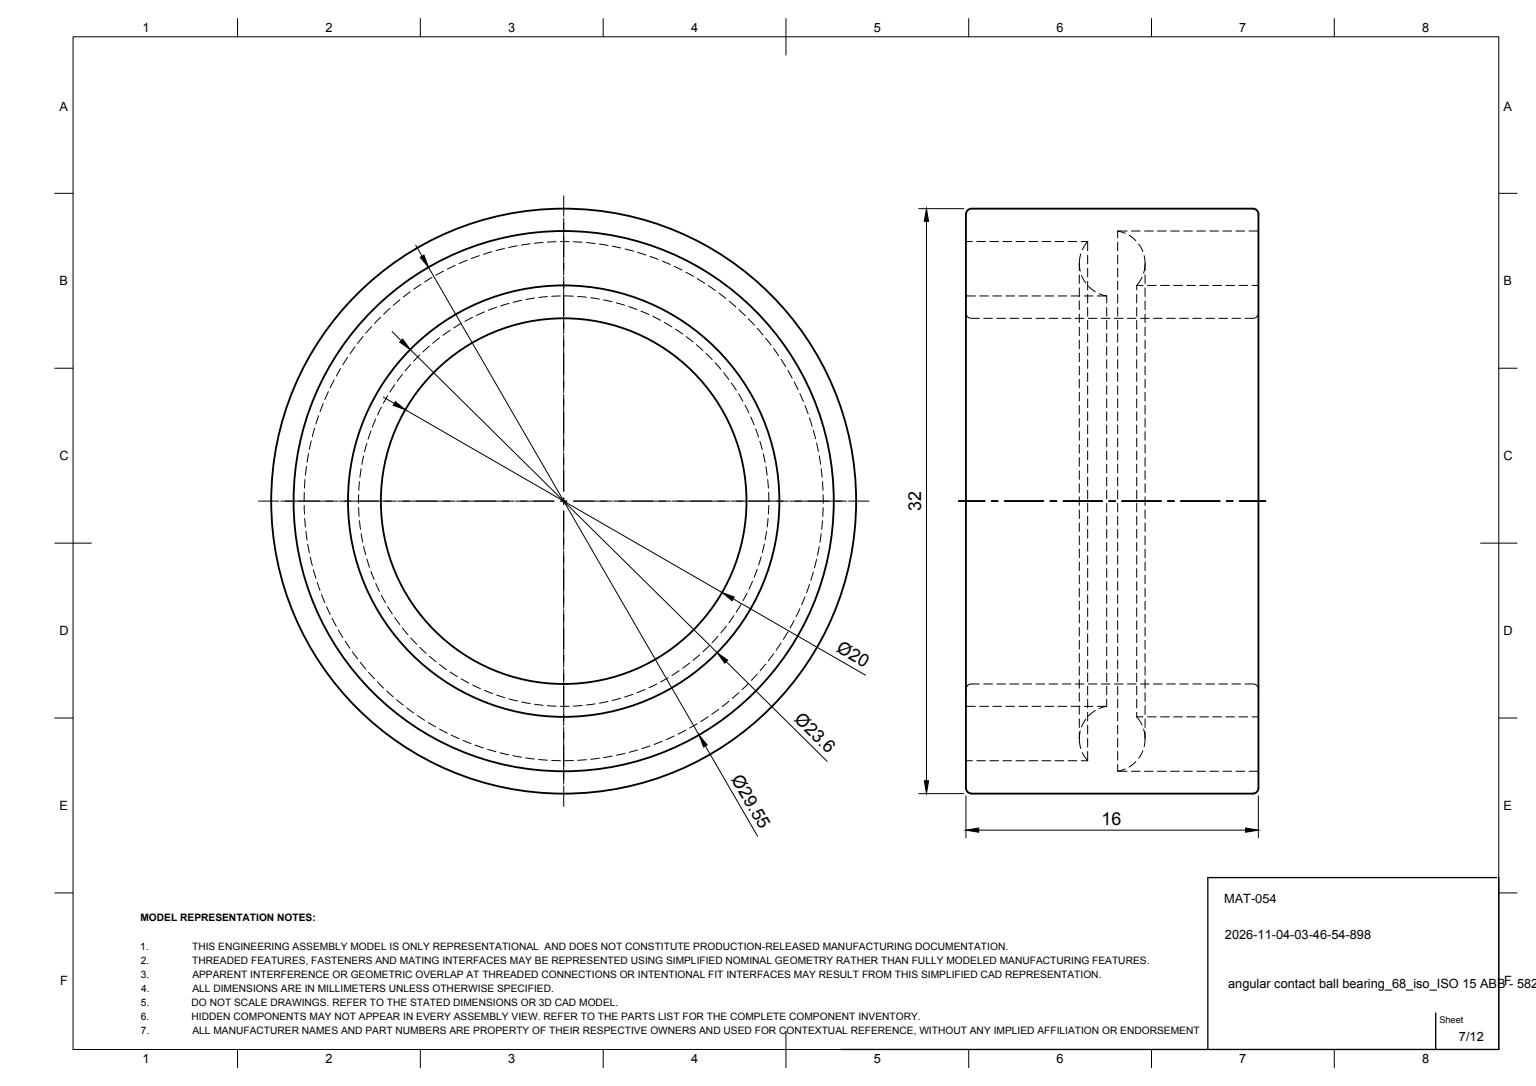
ISO-10303-21;
HEADER;
FILE_DESCRIPTION (('STEP AP214'),
    '1' );
FILE_NAME ('angular contact ball bearing_68_iso_ISO 15 ABB - 5820 - Full,SI,NC,Full_68.step',
    '2026-10-21T17:50:41',
    ( '' ),
    ( '' ),
    'SwSTEP 2.0',
    'SolidWorks 2026',
    '' );
FILE_SCHEMA (( 'AUTOMOTIVE_DESIGN' ));
ENDSEC;

DATA;
#7=EDGE_CURVE ( 'NONE', #6804, #14714, #31558, .T. ) ;
#8=ADVANCED_FACE ( 'NONE', ( #33361 ), #14697, .F. ) ;
#38=PLANE ( 'NONE',  #8347 ) ;
#124=LINE ( 'NONE', #5791, #25297 ) ;
#171=EDGE_CURVE ( 'NONE', #17976, #25124, #32703, .T. ) ;
#186=CARTESIAN_POINT ( 'NONE',  ( 8.000000000000000000, 0.000000000000000000, -14.19999999999999929 ) ) ;
#233=PRODUCT_DEFINITION_FORMATION_WITH_SPECIFIED_SOURCE ( 'ANY', '', #8627, .NOT_KNOWN. ) ;
#246=CARTESIAN_POINT ( 'NONE',  ( 8.000000000000000000, 0.000000000000000000, -15.69999999999999929 ) ) ;
#264=DIRECTION ( 'NONE',  ( 1.000000000000000000, 0.000000000000000000, 0.000000000000000000 ) ) ;
#277=EDGE_CURVE ( 'NONE', #32572, #17435, #29890, .T. ) ;
#329=PRODUCT_DEFINITION ( 'UNKNOWN', '', #233, #29569 ) ;
#379=ORIENTED_EDGE ( 'NONE', *, *, #10888, .T. ) ;
#466=CARTESIAN_POINT ( 'NONE',  ( -0.2989565185775304723, 0.000000000000000000, 0.000000000000000000 ) ) ;
#469=VERTEX_POINT ( 'NONE', #17506 ) ;
#486=AXIS2_PLACEMENT_3D ( 'NONE', #4593, #26151, #10139 ) ;
#668=DIRECTION ( 'NONE',  ( 0.000000000000000000, 0.000000000000000000, -1.000000000000000000 ) ) ;
#744=DIRECTION ( 'NONE',  ( 1.000000000000000000, 0.000000000000000000, 0.000000000000000000 ) ) ;
#769=VERTEX_POINT ( 'NONE', #186 ) ;
#855=EDGE_CURVE ( 'NONE', #32236, #2476, #6011, .T. ) ;
#998=FACE_OUTER_BOUND ( 'NONE', #9441, .T. ) ;
#1009=CARTESIAN_POINT ( 'NONE',  ( -8.000000000000000000, 0.000000000000000000, -15.69999999999999929 ) ) ;
#1061=ORIENTED_EDGE ( 'NONE', *, *, #9092, .F. ) ;
#1105=CARTESIAN_POINT ( 'NONE',  ( -8.000000000000000000, 0.000000000000000000, 0.000000000000000000 ) ) ;
#1140=FACE_OUTER_BOUND ( 'NONE', #5912, .T. ) ;
#1220=CARTESIAN_POINT ( 'NONE',  ( 0.2989565185775198697, 0.000000000000000000, 11.22499999999999787 ) ) ;
#1314=DIRECTION ( 'NONE',  ( 1.000000000000000000, 0.000000000000000000, 0.000000000000000000 ) ) ;
#1338=AXIS2_PLACEMENT_3D ( 'NONE', #14468, #8753, #12149 ) ;
#1470=ORIENTED_EDGE ( 'NONE', *, *, #32484, .T. ) ;
#1474=ORIENTED_EDGE ( 'NONE', *, *, #5517, .F. ) ;
#1512=ORIENTED_EDGE ( 'NONE', *, *, #16791, .T. ) ;
#1621=CIRCLE ( 'NONE', #19248, 16.00000000000000000 ) ;
#1632=EDGE_LOOP ( 'NONE', ( #11200, #2339 ) ) ;
#1652=LINE ( 'NONE', #10193, #28394 ) ;
#1666=CARTESIAN_POINT ( 'NONE',  ( 8.000000000000000000, 0.000000000000000000, 0.000000000000000000 ) ) ;
#1759=DIRECTION ( 'NONE',  ( 0.000000000000000000, 0.000000000000000000, -1.000000000000000000 ) ) ;
#1870=VERTEX_POINT ( 'NONE', #7097 ) ;
#1930=FACE_OUTER_BOUND ( 'NONE', #28195, .T. ) ;
#1931=CARTESIAN_POINT ( 'NONE',  ( -20.63749999999999929, 0.000000000000000000, 0.000000000000000000 ) ) ;
#1947=EDGE_CURVE ( 'NONE', #32236, #1870, #22836, .T. ) ;
#1949=ADVANCED_FACE ( 'NONE', ( #3780 ), #17900, .T. ) ;
#1989=DIRECTION ( 'NONE',  ( 0.000000000000000000, 1.000000000000000000, -1.224646799147353207E-16 ) ) ;
#2151=CYLINDRICAL_SURFACE ( 'NONE', #19584, 16.00000000000000000 ) ;
#2172=ORIENTED_EDGE ( 'NONE', *, *, #16791, .F. ) ;
#2200=DIRECTION ( 'NONE',  ( 0.000000000000000000, 0.000000000000000000, 1.000000000000000000 ) ) ;
#2203=ORIENTED_EDGE ( 'NONE', *, *, #4582, .F. ) ;
#2226=DIRECTION ( 'NONE',  ( 0.000000000000000000, -1.000000000000000000, 0.000000000000000000 ) ) ;
#2240=AXIS2_PLACEMENT_3D ( 'NONE', #7866, #23538, #34222 ) ;
#2314=CYLINDRICAL_SURFACE ( 'NONE', #26398, 11.22499999999999787 ) ;
#2339=ORIENTED_EDGE ( 'NONE', *, *, #22792, .T. ) ;
#2356=DIRECTION ( 'NONE',  ( 0.000000000000000000, 0.000000000000000000, -1.000000000000000000 ) ) ;
#2388=CARTESIAN_POINT ( 'NONE',  ( 8.000000000000000000, 0.000000000000000000, 0.000000000000000000 ) ) ;
#2463=CARTESIAN_POINT ( 'NONE',  ( 7.700000000000000178, 0.000000000000000000, 0.000000000000000000 ) ) ;
#2476=VERTEX_POINT ( 'NONE', #4551 ) ;
#2563=FACE_OUTER_BOUND ( 'NONE', #29011, .T. ) ;
#2569=FACE_OUTER_BOUND ( 'NONE', #17868, .T. ) ;
#2634=AXIS2_PLACEMENT_3D ( 'NONE', #24105, #26962, #27301 ) ;
#2700=CARTESIAN_POINT ( 'NONE',  ( 8.000000000000000000, 0.000000000000000000, 0.000000000000000000 ) ) ;
#2704=DIRECTION ( 'NONE',  ( 0.000000000000000000, 0.000000000000000000, 1.000000000000000000 ) ) ;
#2713=CARTESIAN_POINT ( 'NONE',  ( -1.341640786499875171, 0.000000000000000000, 0.000000000000000000 ) ) ;
#2745=CYLINDRICAL_SURFACE ( 'NONE', #15332, 16.00000000000000000 ) ;
#2757=EDGE_CURVE ( 'NONE', #30850, #6804, #4173, .T. ) ;
#2803=DIRECTION ( 'NONE',  ( 0.000000000000000000, 1.000000000000000000, -1.224646799147353207E-16 ) ) ;
#2837=CARTESIAN_POINT ( 'NONE',  ( 1.341640786499872284, 0.000000000000000000, 0.000000000000000000 ) ) ;
#2846=DIRECTION ( 'NONE',  ( 1.000000000000000000, 0.000000000000000000, 0.000000000000000000 ) ) ;
#2912=CARTESIAN_POINT ( 'NONE',  ( 7.699999999999998401, 0.000000000000000000, 0.000000000000000000 ) ) ;
#2946=DIRECTION ( 'NONE',  ( 1.000000000000000000, 0.000000000000000000, 0.000000000000000000 ) ) ;
#3184=CARTESIAN_POINT ( 'NONE',  ( -7.700000000000000178, 0.000000000000000000, -16.00000000000000000 ) ) ;
#3194=CARTESIAN_POINT ( 'NONE',  ( 7.699999999999998401, 1.959434878635765131E-15, 16.00000000000000000 ) ) ;
#3197=DIRECTION ( 'NONE',  ( 0.000000000000000000, -1.224646799147353454E-16, 1.000000000000000000 ) ) ;
#3275=ORIENTED_EDGE ( 'NONE', *, *, #1947, .F. ) ;
#3330=DIRECTION ( 'NONE',  ( 1.000000000000000000, 0.000000000000000000, 0.000000000000000000 ) ) ;
#3367=DIRECTION ( 'NONE',  ( 0.000000000000000000, 1.224646799147346305E-16, 1.000000000000000000 ) ) ;
#3373=CIRCLE ( 'NONE', #11906, 15.69999999999999929 ) ;
#3511=PLANE ( 'NONE',  #20460 ) ;
#3593=EDGE_CURVE ( 'NONE', #13790, #9326, #20313, .T. ) ;
#3597=TOROIDAL_SURFACE ( 'NONE', #22389, 10.30000000000000071, 0.3000000000000025424 ) ;
#3622=CARTESIAN_POINT ( 'NONE',  ( 7.700000000000001954, 1.243016501134563095E-15, 9.999999999999994671 ) ) ;
#3674=CARTESIAN_POINT ( 'NONE',  ( 8.000000000000000000, 0.000000000000000000, 0.000000000000000000 ) ) ;
#3756=ORIENTED_EDGE ( 'NONE', *, *, #29048, .T. ) ;
#3780=FACE_OUTER_BOUND ( 'NONE', #21252, .T. ) ;
#3795=TOROIDAL_SURFACE ( 'NONE', #27678, 15.69999999999999929, 0.3000000000000007661 ) ;
#3891=TOROIDAL_SURFACE ( 'NONE', #34624, 13.00000000000000000, 1.799999999999999822 ) ;
#3911=TOROIDAL_SURFACE ( 'NONE', #29521, 10.30000000000000071, 0.3000000000000025424 ) ;
#3937=DIRECTION ( 'NONE',  ( 0.000000000000000000, 0.000000000000000000, -1.000000000000000000 ) ) ;
#3990=CIRCLE ( 'NONE', #21637, 1.799999999999999600 ) ;
#4004=FACE_OUTER_BOUND ( 'NONE', #29965, .T. ) ;
#4173=LINE ( 'NONE', #15062, #12299 ) ;
#4194=ORIENTED_EDGE ( 'NONE', *, *, #13037, .T. ) ;
#4241=ADVANCED_FACE ( 'NONE', ( #2563, #31592 ), #7197, .T. ) ;
#4258=TOROIDAL_SURFACE ( 'NONE', #29276, 10.30000000000000071, 0.3000000000000025424 ) ;
#4300=EDGE_LOOP ( 'NONE', ( #16936, #7458, #13111, #5106 ) ) ;
#4312=FACE_OUTER_BOUND ( 'NONE', #33109, .T. ) ;
#4387=CARTESIAN_POINT ( 'NONE',  ( 0.000000000000000000, 0.000000000000000000, 13.00000000000000000 ) ) ;
#4441=CARTESIAN_POINT ( 'NONE',  ( 0.000000000000000000, 1.592040838891559095E-15, -13.00000000000000000 ) ) ;
#4481=ORIENTED_EDGE ( 'NONE', *, *, #29502, .F. ) ;
#4551=CARTESIAN_POINT ( 'NONE',  ( 1.341640786499872284, 1.738998454789241944E-15, -14.20000000000000107 ) ) ;
#4582=EDGE_CURVE ( 'NONE', #22453, #23243, #1652, .T. ) ;
#4593=CARTESIAN_POINT ( 'NONE',  ( 8.000000000000000000, 0.000000000000000000, 0.000000000000000000 ) ) ;
#4623=EDGE_CURVE ( 'NONE', #23243, #30812, #17619, .T. ) ;
#4650=EDGE_LOOP ( 'NONE', ( #32477, #31030, #19102, #11073 ) ) ;
#4704=DIRECTION ( 'NONE',  ( 0.000000000000000000, 0.000000000000000000, -1.000000000000000000 ) ) ;
#4727=DIRECTION ( 'NONE',  ( 1.000000000000000000, 0.000000000000000000, 0.000000000000000000 ) ) ;
#4773=VECTOR ( 'NONE', #4727, 1000.000000000000000 ) ;
#4787=ORIENTED_EDGE ( 'NONE', *, *, #277, .T. ) ;
#4819=ORIENTED_EDGE ( 'NONE', *, *, #29048, .F. ) ;
#4833=DIRECTION ( 'NONE',  ( 1.000000000000000000, 0.000000000000000000, 0.000000000000000000 ) ) ;
#4852=DIRECTION ( 'NONE',  ( 0.000000000000000000, 0.000000000000000000, -1.000000000000000000 ) ) ;
#4894=( NAMED_UNIT ( * ) SI_UNIT ( $, .STERADIAN. ) SOLID_ANGLE_UNIT ( ) );
#4946=CYLINDRICAL_SURFACE ( 'NONE', #12641, 11.80000000000000071 ) ;
#4981=VECTOR ( 'NONE', #744, 1000.000000000000000 ) ;
#5004=CIRCLE ( 'NONE', #24905, 10.30000000000000071 ) ;
#5033=DIRECTION ( 'NONE',  ( 1.000000000000000000, 0.000000000000000000, 0.000000000000000000 ) ) ;
#5086=CARTESIAN_POINT ( 'NONE',  ( -20.63749999999999929, 1.445083222993876839E-15, 11.80000000000000071 ) ) ;
#5106=ORIENTED_EDGE ( 'NONE', *, *, #13037, .F. ) ;
#5174=ORIENTED_EDGE ( 'NONE', *, *, #33517, .F. ) ;
#5178=DIRECTION ( 'NONE',  ( 0.000000000000000000, 0.000000000000000000, -1.000000000000000000 ) ) ;
#5226=DIRECTION ( 'NONE',  ( 1.000000000000000000, 0.000000000000000000, 0.000000000000000000 ) ) ;
#5295=ORIENTED_EDGE ( 'NONE', *, *, #1947, .T. ) ;
#5306=ORIENTED_EDGE ( 'NONE', *, *, #14522, .F. ) ;
#5332=CARTESIAN_POINT ( 'NONE',  ( -8.000000000000000000, 0.000000000000000000, 0.000000000000000000 ) ) ;
#5350=AXIS2_PLACEMENT_3D ( 'NONE', #23000, #33497, #25484 ) ;
#5395=ORIENTED_EDGE ( 'NONE', *, *, #17447, .F. ) ;
#5517=EDGE_CURVE ( 'NONE', #14714, #6804, #6686, .T. ) ;
#5585=DIRECTION ( 'NONE',  ( 0.000000000000000000, 0.000000000000000000, -1.000000000000000000 ) ) ;
#5589=DIRECTION ( 'NONE',  ( 1.000000000000000000, 0.000000000000000000, 0.000000000000000000 ) ) ;
#5616=DIRECTION ( 'NONE',  ( 1.000000000000000000, 0.000000000000000000, 0.000000000000000000 ) ) ;
#5668=ORIENTED_EDGE ( 'NONE', *, *, #22792, .F. ) ;
#5727=STYLED_ITEM('',(#35275),#33706);
#5729=ORIENTED_EDGE ( 'NONE', *, *, #20886, .T. ) ;
#5752=AXIS2_PLACEMENT_3D ( 'NONE', #5332, #16223, #27229 ) ;
#5761=VERTEX_POINT ( 'NONE', #15409 ) ;
#5791=CARTESIAN_POINT ( 'NONE',  ( -20.63749999999999929, 1.374666032042903655E-15, 11.22499999999999787 ) ) ;
#5813=EDGE_CURVE ( 'NONE', #15484, #32236, #12770, .T. ) ;
#5828=CIRCLE ( 'NONE', #18942, 0.3000000000000016542 ) ;
#5912=EDGE_LOOP ( 'NONE', ( #4819, #28442, #12506, #24370 ) ) ;
#6011=CIRCLE ( 'NONE', #35032, 1.799999999999999600 ) ;
#6047=SHAPE_DEFINITION_REPRESENTATION ( #6066, #19821 ) ;
#6052=CARTESIAN_POINT ( 'NONE',  ( 0.2989565185775198697, 0.000000000000000000, 0.000000000000000000 ) ) ;
#6063=LINE ( 'NONE', #13924, #4981 ) ;
#6066=PRODUCT_DEFINITION_SHAPE ( 'NONE', 'NONE',  #329 ) ;
#6110=DIRECTION ( 'NONE',  ( 1.000000000000000000, 0.000000000000000000, 0.000000000000000000 ) ) ;
#6201=DIRECTION ( 'NONE',  ( 0.000000000000000000, 1.000000000000000000, -1.224646799147353207E-16 ) ) ;
#6256=( NAMED_UNIT ( * ) PLANE_ANGLE_UNIT ( ) SI_UNIT ( $, .RADIAN. ) );
#6272=AXIS2_PLACEMENT_3D ( 'NONE', #2388, #13971, #32981 ) ;
#6314=AXIS2_PLACEMENT_3D ( 'NONE', #14281, #24931, #11421 ) ;
#6323=DIRECTION ( 'NONE',  ( 1.000000000000000000, 0.000000000000000000, 0.000000000000000000 ) ) ;
#6375=DIRECTION ( 'NONE',  ( 0.000000000000000000, 0.000000000000000000, -1.000000000000000000 ) ) ;
#6392=ORIENTED_EDGE ( 'NONE', *, *, #9137, .F. ) ;
#6393=CIRCLE ( 'NONE', #21163, 11.79999999999999893 ) ;
#6423=DIRECTION ( 'NONE',  ( 1.000000000000000000, 0.000000000000000000, 0.000000000000000000 ) ) ;
#6595=DIRECTION ( 'NONE',  ( 1.000000000000000000, 0.000000000000000000, 0.000000000000000000 ) ) ;
#6686=CIRCLE ( 'NONE', #17519, 14.77500000000000036 ) ;
#6700=ORIENTED_EDGE ( 'NONE', *, *, #21011, .F. ) ;
#6778=EDGE_CURVE ( 'NONE', #15484, #28564, #124, .T. ) ;
#6804=VERTEX_POINT ( 'NONE', #24847 ) ;
#6851=DIRECTION ( 'NONE',  ( 0.000000000000000000, 0.000000000000000000, 1.000000000000000000 ) ) ;
#6867=ADVANCED_FACE ( 'NONE', ( #4004 ), #32690, .T. ) ;
#6922=DIRECTION ( 'NONE',  ( 1.000000000000000000, 0.000000000000000000, 0.000000000000000000 ) ) ;
#6953=AXIS2_PLACEMENT_3D ( 'NONE', #28762, #23774, #4704 ) ;
#7044=CYLINDRICAL_SURFACE ( 'NONE', #9762, 9.999999999999996447 ) ;
#7063=ORIENTED_EDGE ( 'NONE', *, *, #9331, .F. ) ;
#7086=DIRECTION ( 'NONE',  ( 1.000000000000000000, 0.000000000000000000, 0.000000000000000000 ) ) ;
#7097=CARTESIAN_POINT ( 'NONE',  ( 8.000000000000000000, 0.000000000000000000, -11.22499999999999787 ) ) ;
#7155=CARTESIAN_POINT ( 'NONE',  ( -20.63749999999999574, 0.000000000000000000, 0.000000000000000000 ) ) ;
#7197=PLANE ( 'NONE',  #30658 ) ;
#7243=DIRECTION ( 'NONE',  ( 1.000000000000000000, 0.000000000000000000, 0.000000000000000000 ) ) ;
#7281=EDGE_CURVE ( 'NONE', #23878, #9326, #23633, .T. ) ;
#7393=DIRECTION ( 'NONE',  ( 0.000000000000000000, 0.000000000000000000, -1.000000000000000000 ) ) ;
#7458=ORIENTED_EDGE ( 'NONE', *, *, #33947, .T. ) ;
#7508=CARTESIAN_POINT ( 'NONE',  ( 1.341640786499872284, 0.000000000000000000, 0.000000000000000000 ) ) ;
#7534=DIRECTION ( 'NONE',  ( 1.000000000000000000, 0.000000000000000000, 0.000000000000000000 ) ) ;
#7578=DIRECTION ( 'NONE',  ( 0.000000000000000000, 0.000000000000000000, 1.000000000000000000 ) ) ;
#7612=ORIENTED_EDGE ( 'NONE', *, *, #7281, .F. ) ;
#7665=AXIS2_PLACEMENT_3D ( 'NONE', #17019, #17548, #14516 ) ;
#7702=CARTESIAN_POINT ( 'NONE',  ( 0.2989565185775198697, 1.556832243416072701E-15, -11.22499999999999787 ) ) ;
#7731=DIRECTION ( 'NONE',  ( 0.000000000000000000, 0.000000000000000000, -1.000000000000000000 ) ) ;
#7809=APPLICATION_CONTEXT ( 'automotive_design' ) ;
#7813=AXIS2_PLACEMENT_3D ( 'NONE', #11340, #6323, #8651 ) ;
#7866=CARTESIAN_POINT ( 'NONE',  ( 7.700000000000001954, 0.000000000000000000, 0.000000000000000000 ) ) ;
#7867=DIRECTION ( 'NONE',  ( 0.000000000000000000, 0.000000000000000000, -1.000000000000000000 ) ) ;
#7929=ORIENTED_EDGE ( 'NONE', *, *, #33766, .F. ) ;
#7940=DIRECTION ( 'NONE',  ( -1.000000000000000000, -0.000000000000000000, -0.000000000000000000 ) ) ;
#7994=ORIENTED_EDGE ( 'NONE', *, *, #25214, .T. ) ;
#8003=AXIS2_PLACEMENT_3D ( 'NONE', #10952, #5589, #29819 ) ;
#8066=CIRCLE ( 'NONE', #12634, 9.999999999999998224 ) ;
#8114=LINE ( 'NONE', #5086, #4773 ) ;
#8159=ORIENTED_EDGE ( 'NONE', *, *, #12607, .T. ) ;
#8186=CARTESIAN_POINT ( 'NONE',  ( -20.63749999999999929, 0.000000000000000000, 0.000000000000000000 ) ) ;
#8219=CARTESIAN_POINT ( 'NONE',  ( -8.000000000000000000, 11.79999999999999893, 0.000000000000000000 ) ) ;
#8232=CARTESIAN_POINT ( 'NONE',  ( -20.63749999999999929, 0.000000000000000000, 0.000000000000000000 ) ) ;
#8306=CARTESIAN_POINT ( 'NONE',  ( -7.700000000000000178, 0.000000000000000000, 0.000000000000000000 ) ) ;
#8309=DIRECTION ( 'NONE',  ( 1.000000000000000000, 0.000000000000000000, 0.000000000000000000 ) ) ;
#8347=AXIS2_PLACEMENT_3D ( 'NONE', #8219, #19279, #30114 ) ;
#8352=EDGE_CURVE ( 'NONE', #22453, #21269, #15747, .T. ) ;
#8443=ADVANCED_FACE ( 'NONE', ( #34806 ), #32121, .F. ) ;
#8472=CARTESIAN_POINT ( 'NONE',  ( -7.700000000000000178, 0.000000000000000000, 0.000000000000000000 ) ) ;
#8627=PRODUCT ( 'angular contact ball bearing_68_iso_ISO 15 ABB - 5820 - Full,SI,NC,Full_68', 'angular contact ball bearing_68_iso_ISO 15 ABB - 5820 - Full,SI,NC,Full_68', '', ( #25094 ) ) ;
#8651=DIRECTION ( 'NONE',  ( 0.000000000000000000, 0.000000000000000000, -1.000000000000000000 ) ) ;
#8724=ORIENTED_EDGE ( 'NONE', *, *, #34882, .T. ) ;
#8737=EDGE_LOOP ( 'NONE', ( #34351, #34926 ) ) ;
#8742=DIRECTION ( 'NONE',  ( 0.000000000000000000, 0.000000000000000000, -1.000000000000000000 ) ) ;
#8753=DIRECTION ( 'NONE',  ( 0.000000000000000000, -1.000000000000000000, 0.000000000000000000 ) ) ;
#8771=ORIENTED_EDGE ( 'NONE', *, *, #6778, .F. ) ;
#8856=CARTESIAN_POINT ( 'NONE',  ( 7.700000000000000178, 1.261386203121773722E-15, 10.30000000000000071 ) ) ;
#8889=CARTESIAN_POINT ( 'NONE',  ( 7.700000000000000178, 1.922695474661344271E-15, 15.69999999999999929 ) ) ;
#8915=DIRECTION ( 'NONE',  ( -1.000000000000000000, -0.000000000000000000, -0.000000000000000000 ) ) ;
#8939=AXIS2_PLACEMENT_3D ( 'NONE', #30824, #6423, #17321 ) ;
#8972=CARTESIAN_POINT ( 'NONE',  ( -20.63749999999999574, 0.000000000000000000, 0.000000000000000000 ) ) ;
#9007=DIRECTION ( 'NONE',  ( 0.000000000000000000, 0.000000000000000000, -1.000000000000000000 ) ) ;
#9059=CARTESIAN_POINT ( 'NONE',  ( -7.700000000000000178, 0.000000000000000000, 0.000000000000000000 ) ) ;
#9092=EDGE_CURVE ( 'NONE', #5761, #30633, #17839, .T. ) ;
#9137=EDGE_CURVE ( 'NONE', #5761, #469, #16938, .T. ) ;
#9319=DIRECTION ( 'NONE',  ( 1.000000000000000000, 0.000000000000000000, 0.000000000000000000 ) ) ;
#9326=VERTEX_POINT ( 'NONE', #3194 ) ;
#9331=EDGE_CURVE ( 'NONE', #469, #5761, #6393, .T. ) ;
#9441=EDGE_LOOP ( 'NONE', ( #11859, #34213, #13046, #18356 ) ) ;
#9495=ORIENTED_EDGE ( 'NONE', *, *, #17447, .T. ) ;
#9525=EDGE_LOOP ( 'NONE', ( #4787, #8724, #10418, #34158 ) ) ;
#9653=ORIENTED_EDGE ( 'NONE', *, *, #18373, .F. ) ;
#9667=DIRECTION ( 'NONE',  ( 0.000000000000000000, 0.000000000000000000, -1.000000000000000000 ) ) ;
#9728=ADVANCED_FACE ( 'NONE', ( #14262 ), #25090, .T. ) ;
#9762=AXIS2_PLACEMENT_3D ( 'NONE', #28429, #28774, #7393 ) ;
#9811=CIRCLE ( 'NONE', #6953, 0.3000000000000016542 ) ;
#9838=LINE ( 'NONE', #33697, #11415 ) ;
#9871=EDGE_CURVE ( 'NONE', #12372, #21269, #5004, .T. ) ;
#9894=ORIENTED_EDGE ( 'NONE', *, *, #171, .F. ) ;
#9902=ORIENTED_EDGE ( 'NONE', *, *, #7, .F. ) ;
#9903=FACE_OUTER_BOUND ( 'NONE', #34611, .T. ) ;
#9958=CARTESIAN_POINT ( 'NONE',  ( -8.000000000000000000, 0.000000000000000000, 0.000000000000000000 ) ) ;
#10045=VERTEX_POINT ( 'NONE', #18861 ) ;
#10070=ORIENTED_EDGE ( 'NONE', *, *, #17795, .T. ) ;
#10139=DIRECTION ( 'NONE',  ( 0.000000000000000000, 0.000000000000000000, -1.000000000000000000 ) ) ;
#10150=ORIENTED_EDGE ( 'NONE', *, *, #21782, .T. ) ;
#10158=DIRECTION ( 'NONE',  ( 0.000000000000000000, 0.000000000000000000, -1.000000000000000000 ) ) ;
#10193=CARTESIAN_POINT ( 'NONE',  ( -20.63749999999999929, 0.000000000000000000, -9.999999999999996447 ) ) ;
#10288=ORIENTED_EDGE ( 'NONE', *, *, #29502, .T. ) ;
#10303=FACE_OUTER_BOUND ( 'NONE', #4300, .T. ) ;
#10353=ADVANCED_FACE ( 'NONE', ( #29662 ), #3891, .T. ) ;
#10404=DIRECTION ( 'NONE',  ( 1.000000000000000000, 0.000000000000000000, 0.000000000000000000 ) ) ;
#10418=ORIENTED_EDGE ( 'NONE', *, *, #4623, .F. ) ;
#10452=CIRCLE ( 'NONE', #34899, 15.69999999999999929 ) ;
#10530=ADVANCED_FACE ( 'NONE', ( #998 ), #3911, .T. ) ;
#10585=LINE ( 'NONE', #23572, #22995 ) ;
#10716=CARTESIAN_POINT ( 'NONE',  ( -7.700000000000000178, 1.959434878635765131E-15, 16.00000000000000000 ) ) ;
#10746=CYLINDRICAL_SURFACE ( 'NONE', #29146, 11.80000000000000071 ) ;
#10766=CARTESIAN_POINT ( 'NONE',  ( -20.63749999999999574, 0.000000000000000000, -14.20000000000000107 ) ) ;
#10783=ORIENTED_EDGE ( 'NONE', *, *, #14522, .T. ) ;
#10861=MECHANICAL_DESIGN_GEOMETRIC_PRESENTATION_REPRESENTATION('',(#5727),#18268);
#10888=EDGE_CURVE ( 'NONE', #28564, #1870, #29393, .T. ) ;
#10908=CIRCLE ( 'NONE', #16052, 0.3000000000000016542 ) ;
#10952=CARTESIAN_POINT ( 'NONE',  ( -8.000000000000000000, 0.000000000000000000, 0.000000000000000000 ) ) ;
#10955=CIRCLE ( 'NONE', #33689, 0.3000000000000016542 ) ;
#11008=CIRCLE ( 'NONE', #34877, 16.00000000000000000 ) ;
#11073=ORIENTED_EDGE ( 'NONE', *, *, #8352, .F. ) ;
#11126=DIRECTION ( 'NONE',  ( 0.000000000000000000, 0.000000000000000000, -1.000000000000000000 ) ) ;
#11200=ORIENTED_EDGE ( 'NONE', *, *, #33766, .T. ) ;
#11255=TOROIDAL_SURFACE ( 'NONE', #31151, 15.69999999999999929, 0.3000000000000007661 ) ;
#11285=ORIENTED_EDGE ( 'NONE', *, *, #9137, .T. ) ;
#11340=CARTESIAN_POINT ( 'NONE',  ( -20.63749999999999574, 0.000000000000000000, 0.000000000000000000 ) ) ;
#11346=FACE_OUTER_BOUND ( 'NONE', #22853, .T. ) ;
#11358=ORIENTED_EDGE ( 'NONE', *, *, #7, .T. ) ;
#11372=EDGE_LOOP ( 'NONE', ( #19791, #18009, #10783, #30053 ) ) ;
#11413=DIRECTION ( 'NONE',  ( 0.000000000000000000, 0.000000000000000000, 1.000000000000000000 ) ) ;
#11415=VECTOR ( 'NONE', #9319, 1000.000000000000000 ) ;
#11421=DIRECTION ( 'NONE',  ( 0.000000000000000000, 0.000000000000000000, 1.000000000000000000 ) ) ;
#11466=DIRECTION ( 'NONE',  ( 1.000000000000000000, 0.000000000000000000, 0.000000000000000000 ) ) ;
#11522=ADVANCED_FACE ( 'NONE', ( #14189 ), #14726, .F. ) ;
#11527=CIRCLE ( 'NONE', #34824, 16.00000000000000000 ) ;
#11699=DIRECTION ( 'NONE',  ( 0.000000000000000000, 0.000000000000000000, 1.000000000000000000 ) ) ;
#11750=ORIENTED_EDGE ( 'NONE', *, *, #25952, .T. ) ;
#11789=EDGE_CURVE ( 'NONE', #2476, #769, #32284, .T. ) ;
#11816=( NAMED_UNIT ( * ) SI_UNIT ( $, .STERADIAN. ) SOLID_ANGLE_UNIT ( ) );
#11859=ORIENTED_EDGE ( 'NONE', *, *, #28498, .F. ) ;
#11906=AXIS2_PLACEMENT_3D ( 'NONE', #29629, #5226, #34804 ) ;
#11989=DIRECTION ( 'NONE',  ( 0.000000000000000000, 0.000000000000000000, -1.000000000000000000 ) ) ;
#12004=CYLINDRICAL_SURFACE ( 'NONE', #22813, 14.20000000000000107 ) ;
#12149=DIRECTION ( 'NONE',  ( 0.000000000000000000, 0.000000000000000000, -1.000000000000000000 ) ) ;
#12158=EDGE_CURVE ( 'NONE', #20178, #13790, #1621, .T. ) ;
#12279=AXIS2_PLACEMENT_3D ( 'NONE', #1666, #34061, #23892 ) ;
#12299=VECTOR ( 'NONE', #33384, 1000.000000000000000 ) ;
#12321=CARTESIAN_POINT ( 'NONE',  ( -20.63749999999999929, 0.000000000000000000, -11.80000000000000071 ) ) ;
#12372=VERTEX_POINT ( 'NONE', #17623 ) ;
#12506=ORIENTED_EDGE ( 'NONE', *, *, #11789, .T. ) ;
#12544=CARTESIAN_POINT ( 'NONE',  ( -7.700000000000000178, 1.261386203121773722E-15, 10.30000000000000071 ) ) ;
#12590=AXIS2_PLACEMENT_3D ( 'NONE', #4441, #20318, #17662 ) ;
#12601=DIRECTION ( 'NONE',  ( 0.000000000000000000, -1.000000000000000000, 0.000000000000000000 ) ) ;
#12607=EDGE_CURVE ( 'NONE', #29267, #16011, #14737, .T. ) ;
#12634=AXIS2_PLACEMENT_3D ( 'NONE', #8306, #5616, #16873 ) ;
#12641=AXIS2_PLACEMENT_3D ( 'NONE', #1931, #32354, #29168 ) ;
#12753=DIRECTION ( 'NONE',  ( -0.000000000000000000, 0.000000000000000000, 1.000000000000000000 ) ) ;
#12767=EDGE_LOOP ( 'NONE', ( #32048, #28767, #24933, #2203 ) ) ;
#12770=CIRCLE ( 'NONE', #33202, 11.22499999999999787 ) ;
#12772=CARTESIAN_POINT ( 'NONE',  ( -20.63749999999999574, 1.738998454789241549E-15, 14.20000000000000107 ) ) ;
#12789=ADVANCED_FACE ( 'NONE', ( #11346 ), #13575, .T. ) ;
#12887=ADVANCED_FACE ( 'NONE', ( #28756, #20753 ), #17749, .T. ) ;
#12910=EDGE_LOOP ( 'NONE', ( #25875, #33507 ) ) ;
#12965=FACE_OUTER_BOUND ( 'NONE', #23359, .T. ) ;
#13012=CARTESIAN_POINT ( 'NONE',  ( -7.700000000000000178, 1.224646799147353059E-15, 9.999999999999998224 ) ) ;
#13037=EDGE_CURVE ( 'NONE', #25124, #17976, #3373, .T. ) ;
#13046=ORIENTED_EDGE ( 'NONE', *, *, #8352, .T. ) ;
#13070=ADVANCED_FACE ( 'NONE', ( #2569 ), #2745, .T. ) ;
#13073=DIRECTION ( 'NONE',  ( 1.000000000000000000, 0.000000000000000000, 0.000000000000000000 ) ) ;
#13101=EDGE_CURVE ( 'NONE', #17435, #32572, #13596, .T. ) ;
#13111=ORIENTED_EDGE ( 'NONE', *, *, #25853, .T. ) ;
#13185=ORIENTED_EDGE ( 'NONE', *, *, #25983, .T. ) ;
#13336=FACE_OUTER_BOUND ( 'NONE', #25393, .T. ) ;
#13344=DIRECTION ( 'NONE',  ( 1.000000000000000000, 0.000000000000000000, 0.000000000000000000 ) ) ;
#13385=ADVANCED_FACE ( 'NONE', ( #17434, #22394 ), #3511, .T. ) ;
#13575=TOROIDAL_SURFACE ( 'NONE', #26649, 13.00000000000000000, 1.799999999999999822 ) ;
#13596=CIRCLE ( 'NONE', #28389, 10.30000000000000071 ) ;
#13641=AXIS2_PLACEMENT_3D ( 'NONE', #23154, #31317, #28652 ) ;
#13790=VERTEX_POINT ( 'NONE', #10716 ) ;
#13792=DIRECTION ( 'NONE',  ( 0.000000000000000000, 0.000000000000000000, -1.000000000000000000 ) ) ;
#13805=AXIS2_PLACEMENT_3D ( 'NONE', #19407, #13887, #29907 ) ;
#13850=DIRECTION ( 'NONE',  ( 0.000000000000000000, 1.224646799147359124E-16, 1.000000000000000000 ) ) ;
#13887=DIRECTION ( 'NONE',  ( 1.000000000000000000, 0.000000000000000000, 0.000000000000000000 ) ) ;
#13924=CARTESIAN_POINT ( 'NONE',  ( -20.63749999999999929, 1.224646799147352862E-15, 9.999999999999996447 ) ) ;
#13967=CARTESIAN_POINT ( 'NONE',  ( 8.000000000000000000, 1.738998454789241155E-15, 14.19999999999999929 ) ) ;
#13971=DIRECTION ( 'NONE',  ( 1.000000000000000000, 0.000000000000000000, 0.000000000000000000 ) ) ;
#13988=EDGE_LOOP ( 'NONE', ( #9653, #8159, #21922, #20482 ) ) ;
#14123=EDGE_CURVE ( 'NONE', #28125, #30633, #27860, .T. ) ;
#14145=LINE ( 'NONE', #12772, #17682 ) ;
#14171=ORIENTED_EDGE ( 'NONE', *, *, #11789, .F. ) ;
#14189=FACE_OUTER_BOUND ( 'NONE', #19126, .T. ) ;
#14262=FACE_OUTER_BOUND ( 'NONE', #16003, .T. ) ;
#14281=CARTESIAN_POINT ( 'NONE',  ( 0.2989565185775198697, 0.000000000000000000, 0.000000000000000000 ) ) ;
#14468=CARTESIAN_POINT ( 'NONE',  ( 7.700000000000000178, 0.000000000000000000, -15.69999999999999929 ) ) ;
#14472=CARTESIAN_POINT ( 'NONE',  ( 8.000000000000003553, 0.000000000000000000, -10.30000000000000071 ) ) ;
#14498=EDGE_LOOP ( 'NONE', ( #6392, #7063 ) ) ;
#14516=DIRECTION ( 'NONE',  ( 0.000000000000000000, 0.000000000000000000, -1.000000000000000000 ) ) ;
#14522=EDGE_CURVE ( 'NONE', #6804, #28125, #3990, .T. ) ;
#14539=AXIS2_PLACEMENT_3D ( 'NONE', #24282, #19634, #5585 ) ;
#14553=DIRECTION ( 'NONE',  ( -1.000000000000000000, -0.000000000000000000, -0.000000000000000000 ) ) ;
#14558=CARTESIAN_POINT ( 'NONE',  ( 8.000000000000000000, 1.941065176648554701E-15, 15.69999999999999929 ) ) ;
#14640=DIRECTION ( 'NONE',  ( 0.000000000000000000, -1.000000000000000000, 0.000000000000000000 ) ) ;
#14679=ORIENTED_EDGE ( 'NONE', *, *, #9331, .T. ) ;
#14697=CYLINDRICAL_SURFACE ( 'NONE', #7665, 14.77500000000000036 ) ;
#14714=VERTEX_POINT ( 'NONE', #17041 ) ;
#14726=CYLINDRICAL_SURFACE ( 'NONE', #7813, 14.20000000000000107 ) ;
#14737=CIRCLE ( 'NONE', #34605, 15.69999999999999929 ) ;
#14748=DIRECTION ( 'NONE',  ( 1.000000000000000000, 0.000000000000000000, 0.000000000000000000 ) ) ;
#15008=AXIS2_PLACEMENT_3D ( 'NONE', #1105, #23687, #15338 ) ;
#15062=CARTESIAN_POINT ( 'NONE',  ( -20.63749999999999574, 1.809415645740214338E-15, 14.77500000000000036 ) ) ;
#15183=ORIENTED_EDGE ( 'NONE', *, *, #2757, .T. ) ;
#15223=ORIENTED_EDGE ( 'NONE', *, *, #10888, .F. ) ;
#15332=AXIS2_PLACEMENT_3D ( 'NONE', #15951, #24276, #13792 ) ;
#15338=DIRECTION ( 'NONE',  ( 0.000000000000000000, 0.000000000000000000, -1.000000000000000000 ) ) ;
#15391=DIRECTION ( 'NONE',  ( 0.000000000000000000, 0.000000000000000000, -1.000000000000000000 ) ) ;
#15409=CARTESIAN_POINT ( 'NONE',  ( -8.000000000000000000, 0.000000000000000000, -11.79999999999999893 ) ) ;
#15437=AXIS2_PLACEMENT_3D ( 'NONE', #25640, #6595, #17495 ) ;
#15484=VERTEX_POINT ( 'NONE', #1220 ) ;
#15516=FACE_OUTER_BOUND ( 'NONE', #20039, .T. ) ;
#15536=ORIENTED_EDGE ( 'NONE', *, *, #15862, .F. ) ;
#15747=CIRCLE ( 'NONE', #19147, 0.3000000000000016542 ) ;
#15846=CARTESIAN_POINT ( 'NONE',  ( -8.000000000000001776, 0.000000000000000000, -10.30000000000000071 ) ) ;
#15862=EDGE_CURVE ( 'NONE', #22453, #29721, #8066, .T. ) ;
#15932=DIRECTION ( 'NONE',  ( 0.000000000000000000, 0.000000000000000000, -1.000000000000000000 ) ) ;
#15951=CARTESIAN_POINT ( 'NONE',  ( -20.63749999999999574, 0.000000000000000000, 0.000000000000000000 ) ) ;
#15971=ORIENTED_EDGE ( 'NONE', *, *, #18373, .T. ) ;
#15987=DIRECTION ( 'NONE',  ( 0.000000000000000000, 0.000000000000000000, -1.000000000000000000 ) ) ;
#16003=EDGE_LOOP ( 'NONE', ( #8771, #4481, #5295, #15223 ) ) ;
#16011=VERTEX_POINT ( 'NONE', #1009 ) ;
#16047=CARTESIAN_POINT ( 'NONE',  ( 7.699999999999998401, 0.000000000000000000, -16.00000000000000000 ) ) ;
#16052=AXIS2_PLACEMENT_3D ( 'NONE', #8856, #2803, #13850 ) ;
#16098=ORIENTED_EDGE ( 'NONE', *, *, #16365, .T. ) ;
#16116=DIRECTION ( 'NONE',  ( 1.000000000000000000, 0.000000000000000000, 0.000000000000000000 ) ) ;
#16219=DIRECTION ( 'NONE',  ( 0.000000000000000000, 0.000000000000000000, 1.000000000000000000 ) ) ;
#16223=DIRECTION ( 'NONE',  ( 1.000000000000000000, 0.000000000000000000, 0.000000000000000000 ) ) ;
#16365=EDGE_CURVE ( 'NONE', #19238, #769, #21635, .T. ) ;
#16377=ADVANCED_FACE ( 'NONE', ( #1140 ), #12004, .F. ) ;
#16665=ORIENTED_EDGE ( 'NONE', *, *, #9871, .T. ) ;
#16693=CIRCLE ( 'NONE', #1338, 0.3000000000000016542 ) ;
#16791=EDGE_CURVE ( 'NONE', #15484, #26364, #24067, .T. ) ;
#16873=DIRECTION ( 'NONE',  ( 0.000000000000000000, 0.000000000000000000, -1.000000000000000000 ) ) ;
#16936=ORIENTED_EDGE ( 'NONE', *, *, #31141, .F. ) ;
#16938=CIRCLE ( 'NONE', #8939, 11.79999999999999893 ) ;
#17019=CARTESIAN_POINT ( 'NONE',  ( -20.63749999999999574, 0.000000000000000000, 0.000000000000000000 ) ) ;
#17036=ORIENTED_EDGE ( 'NONE', *, *, #12158, .F. ) ;
#17041=CARTESIAN_POINT ( 'NONE',  ( -0.2989565185775304723, 1.809415645740214338E-15, -14.77500000000000036 ) ) ;
#17071=CARTESIAN_POINT ( 'NONE',  ( 8.000000000000001776, 10.30000000000000071, 0.000000000000000000 ) ) ;
#17079=ORIENTED_EDGE ( 'NONE', *, *, #171, .T. ) ;
#17157=CIRCLE ( 'NONE', #6314, 11.22499999999999787 ) ;
#17234=( GEOMETRIC_REPRESENTATION_CONTEXT ( 3 ) GLOBAL_UNCERTAINTY_ASSIGNED_CONTEXT ( ( #17805 ) ) GLOBAL_UNIT_ASSIGNED_CONTEXT ( ( #19822, #6256, #11816 ) ) REPRESENTATION_CONTEXT ( 'NONE', 'WORKASPACE' ) );
#17308=CARTESIAN_POINT ( 'NONE',  ( -20.63749999999999574, 1.959434878635765131E-15, 16.00000000000000000 ) ) ;
#17321=DIRECTION ( 'NONE',  ( 0.000000000000000000, 0.000000000000000000, -1.000000000000000000 ) ) ;
#17381=ORIENTED_EDGE ( 'NONE', *, *, #34882, .F. ) ;
#17434=FACE_OUTER_BOUND ( 'NONE', #23390, .T. ) ;
#17435=VERTEX_POINT ( 'NONE', #31794 ) ;
#17447=EDGE_CURVE ( 'NONE', #469, #28125, #8114, .T. ) ;
#17495=DIRECTION ( 'NONE',  ( 0.000000000000000000, 0.000000000000000000, -1.000000000000000000 ) ) ;
#17506=CARTESIAN_POINT ( 'NONE',  ( -8.000000000000000000, 1.445083222993876839E-15, 11.79999999999999893 ) ) ;
#17519=AXIS2_PLACEMENT_3D ( 'NONE', #466, #32839, #30899 ) ;
#17527=EDGE_LOOP ( 'NONE', ( #11750, #16665 ) ) ;
#17548=DIRECTION ( 'NONE',  ( 1.000000000000000000, 0.000000000000000000, 0.000000000000000000 ) ) ;
#17619=CIRCLE ( 'NONE', #2240, 9.999999999999994671 ) ;
#17623=CARTESIAN_POINT ( 'NONE',  ( -8.000000000000001776, 1.261386203121773722E-15, 10.30000000000000071 ) ) ;
#17638=CARTESIAN_POINT ( 'NONE',  ( 7.700000000000000178, 0.000000000000000000, 0.000000000000000000 ) ) ;
#17662=DIRECTION ( 'NONE',  ( 0.000000000000000000, -1.224646799147353454E-16, 1.000000000000000000 ) ) ;
#17682=VECTOR ( 'NONE', #11466, 1000.000000000000000 ) ;
#17704=DIRECTION ( 'NONE',  ( 1.000000000000000000, 0.000000000000000000, 0.000000000000000000 ) ) ;
#17714=TOROIDAL_SURFACE ( 'NONE', #15437, 10.30000000000000071, 0.3000000000000025424 ) ;
#17749=PLANE ( 'NONE',  #20435 ) ;
#17785=AXIS2_PLACEMENT_3D ( 'NONE', #20081, #14748, #15391 ) ;
#17795=EDGE_CURVE ( 'NONE', #20178, #23878, #10585, .T. ) ;
#17805=UNCERTAINTY_MEASURE_WITH_UNIT (LENGTH_MEASURE( 1.000000000000000082E-05 ), #19822, 'distance_accuracy_value', 'NONE');
#17839=LINE ( 'NONE', #12321, #27117 ) ;
#17845=DIRECTION ( 'NONE',  ( 0.000000000000000000, 0.000000000000000000, -1.000000000000000000 ) ) ;
#17868=EDGE_LOOP ( 'NONE', ( #27198, #13185, #10070, #20481 ) ) ;
#17900=TOROIDAL_SURFACE ( 'NONE', #19590, 15.69999999999999929, 0.3000000000000007661 ) ;
#17904=DIRECTION ( 'NONE',  ( 0.000000000000000000, 1.000000000000000000, -1.224646799147353207E-16 ) ) ;
#17937=AXIS2_PLACEMENT_3D ( 'NONE', #26372, #1989, #19611 ) ;
#17976=VERTEX_POINT ( 'NONE', #246 ) ;
#18009=ORIENTED_EDGE ( 'NONE', *, *, #5517, .T. ) ;
#18100=DIRECTION ( 'NONE',  ( 0.000000000000000000, 0.000000000000000000, -1.000000000000000000 ) ) ;
#18199=CARTESIAN_POINT ( 'NONE',  ( -7.700000000000000178, 0.000000000000000000, -15.69999999999999929 ) ) ;
#18268=( GEOMETRIC_REPRESENTATION_CONTEXT ( 3 ) GLOBAL_UNCERTAINTY_ASSIGNED_CONTEXT ( ( #19639 ) ) GLOBAL_UNIT_ASSIGNED_CONTEXT ( ( #32474, #21286, #4894 ) ) REPRESENTATION_CONTEXT ( 'NONE', 'WORKASPACE' ) );
#18356=ORIENTED_EDGE ( 'NONE', *, *, #9871, .F. ) ;
#18373=EDGE_CURVE ( 'NONE', #29267, #13790, #21894, .T. ) ;
#18394=CARTESIAN_POINT ( 'NONE',  ( -7.700000000000000178, 0.000000000000000000, 0.000000000000000000 ) ) ;
#18437=CARTESIAN_POINT ( 'NONE',  ( 8.000000000000000000, 15.69999999999999929, 0.000000000000000000 ) ) ;
#18580=CARTESIAN_POINT ( 'NONE',  ( 0.000000000000000000, 0.000000000000000000, 13.00000000000000000 ) ) ;
#18589=DIRECTION ( 'NONE',  ( 1.000000000000000000, 0.000000000000000000, 0.000000000000000000 ) ) ;
#18791=DIRECTION ( 'NONE',  ( 0.000000000000000000, 0.000000000000000000, -1.000000000000000000 ) ) ;
#18840=ORIENTED_EDGE ( 'NONE', *, *, #14123, .F. ) ;
#18848=AXIS2_PLACEMENT_3D ( 'NONE', #12544, #17904, #22878 ) ;
#18861=CARTESIAN_POINT ( 'NONE',  ( -8.000000000000000000, 0.000000000000000000, -14.77499999999999858 ) ) ;
#18942=AXIS2_PLACEMENT_3D ( 'NONE', #18199, #26175, #3937 ) ;
#18963=EDGE_LOOP ( 'NONE', ( #11358, #31098, #1470, #5306 ) ) ;
#19102=ORIENTED_EDGE ( 'NONE', *, *, #25952, .F. ) ;
#19126=EDGE_LOOP ( 'NONE', ( #33333, #3756, #16098, #14171 ) ) ;
#19147=AXIS2_PLACEMENT_3D ( 'NONE', #26607, #2226, #18791 ) ;
#19155=FACE_OUTER_BOUND ( 'NONE', #4650, .T. ) ;
#19188=DIRECTION ( 'NONE',  ( 1.000000000000000000, 0.000000000000000000, 0.000000000000000000 ) ) ;
#19238=VERTEX_POINT ( 'NONE', #13967 ) ;
#19248=AXIS2_PLACEMENT_3D ( 'NONE', #18394, #26380, #5178 ) ;
#19279=DIRECTION ( 'NONE',  ( -1.000000000000000000, 0.000000000000000000, -0.000000000000000000 ) ) ;
#19407=CARTESIAN_POINT ( 'NONE',  ( -7.700000000000000178, 0.000000000000000000, 0.000000000000000000 ) ) ;
#19584=AXIS2_PLACEMENT_3D ( 'NONE', #21021, #20842, #17845 ) ;
#19590=AXIS2_PLACEMENT_3D ( 'NONE', #28823, #25492, #11989 ) ;
#19611=DIRECTION ( 'NONE',  ( 0.000000000000000000, 1.224646799147346305E-16, 1.000000000000000000 ) ) ;
#19634=DIRECTION ( 'NONE',  ( -1.000000000000000000, -0.000000000000000000, -0.000000000000000000 ) ) ;
#19639=UNCERTAINTY_MEASURE_WITH_UNIT (LENGTH_MEASURE( 1.000000000000000082E-05 ), #32474, 'distance_accuracy_value', 'NONE');
#19791=ORIENTED_EDGE ( 'NONE', *, *, #29582, .F. ) ;
#19821=SHAPE_REPRESENTATION ( 'angular contact ball bearing_68_iso_ISO 15 ABB - 5820 - Full,SI,NC,Full_68', ( #28566 ), #17234 ) ;
#19822=( LENGTH_UNIT ( ) NAMED_UNIT ( * ) SI_UNIT ( .MILLI., .METRE. ) );
#19923=DIRECTION ( 'NONE',  ( 1.000000000000000000, 0.000000000000000000, 0.000000000000000000 ) ) ;
#19995=ORIENTED_EDGE ( 'NONE', *, *, #4582, .T. ) ;
#20021=TOROIDAL_SURFACE ( 'NONE', #24530, 15.69999999999999929, 0.3000000000000007661 ) ;
#20039=EDGE_LOOP ( 'NONE', ( #25202, #32841, #7612, #34086 ) ) ;
#20081=CARTESIAN_POINT ( 'NONE',  ( 7.700000000000001954, 0.000000000000000000, 0.000000000000000000 ) ) ;
#20178=VERTEX_POINT ( 'NONE', #3184 ) ;
#20224=AXIS2_PLACEMENT_3D ( 'NONE', #32262, #18589, #2356 ) ;
#20240=CARTESIAN_POINT ( 'NONE',  ( 0.000000000000000000, 0.000000000000000000, 0.000000000000000000 ) ) ;
#20242=AXIS2_PLACEMENT_3D ( 'NONE', #2912, #6110, #11126 ) ;
#20313=LINE ( 'NONE', #17308, #23218 ) ;
#20318=DIRECTION ( 'NONE',  ( -0.000000000000000000, 1.000000000000000000, 1.224646799147353207E-16 ) ) ;
#20420=DIRECTION ( 'NONE',  ( -0.000000000000000000, 1.000000000000000000, 1.224646799147353207E-16 ) ) ;
#20426=ADVANCED_FACE ( 'NONE', ( #25242 ), #3795, .T. ) ;
#20435=AXIS2_PLACEMENT_3D ( 'NONE', #21091, #28587, #12753 ) ;
#20460=AXIS2_PLACEMENT_3D ( 'NONE', #17071, #30582, #25042 ) ;
#20481=ORIENTED_EDGE ( 'NONE', *, *, #33947, .F. ) ;
#20482=ORIENTED_EDGE ( 'NONE', *, *, #25983, .F. ) ;
#20689=ORIENTED_EDGE ( 'NONE', *, *, #5813, .T. ) ;
#20753=FACE_OUTER_BOUND ( 'NONE', #8737, .T. ) ;
#20813=ADVANCED_FACE ( 'NONE', ( #4312 ), #23208, .F. ) ;
#20842=DIRECTION ( 'NONE',  ( 1.000000000000000000, 0.000000000000000000, 0.000000000000000000 ) ) ;
#20886=EDGE_CURVE ( 'NONE', #26364, #2476, #31660, .T. ) ;
#21003=ORIENTED_EDGE ( 'NONE', *, *, #16365, .F. ) ;
#21011=EDGE_CURVE ( 'NONE', #29721, #30812, #6063, .T. ) ;
#21021=CARTESIAN_POINT ( 'NONE',  ( -20.63749999999999574, 0.000000000000000000, 0.000000000000000000 ) ) ;
#21091=CARTESIAN_POINT ( 'NONE',  ( -8.000000000000000000, 14.77499999999999858, 0.000000000000000000 ) ) ;
#21113=CIRCLE ( 'NONE', #12590, 1.799999999999999600 ) ;
#21120=CIRCLE ( 'NONE', #5752, 14.77499999999999858 ) ;
#21163=AXIS2_PLACEMENT_3D ( 'NONE', #23901, #5033, #15932 ) ;
#21184=DIRECTION ( 'NONE',  ( 1.000000000000000000, 0.000000000000000000, 0.000000000000000000 ) ) ;
#21229=APPLICATION_CONTEXT ( 'automotive_design' ) ;
#21248=ADVANCED_FACE ( 'NONE', ( #10303 ), #11255, .T. ) ;
#21252=EDGE_LOOP ( 'NONE', ( #22324, #26243, #9894, #25661 ) ) ;
#21269=VERTEX_POINT ( 'NONE', #15846 ) ;
#21286=( NAMED_UNIT ( * ) PLANE_ANGLE_UNIT ( ) SI_UNIT ( $, .RADIAN. ) );
#21411=AXIS2_PLACEMENT_3D ( 'NONE', #2837, #21184, #16219 ) ;
#21419=ADVANCED_FACE ( 'NONE', ( #29764, #24411 ), #38, .T. ) ;
#21544=ORIENTED_EDGE ( 'NONE', *, *, #5813, .F. ) ;
#21573=ORIENTED_EDGE ( 'NONE', *, *, #4623, .T. ) ;
#21635=CIRCLE ( 'NONE', #6272, 14.19999999999999929 ) ;
#21637=AXIS2_PLACEMENT_3D ( 'NONE', #4387, #12601, #31455 ) ;
#21647=AXIS2_PLACEMENT_3D ( 'NONE', #2700, #4833, #7867 ) ;
#21782=EDGE_CURVE ( 'NONE', #2476, #26364, #23695, .T. ) ;
#21894=CIRCLE ( 'NONE', #17937, 0.3000000000000016542 ) ;
#21922=ORIENTED_EDGE ( 'NONE', *, *, #34316, .T. ) ;
#21953=ORIENTED_EDGE ( 'NONE', *, *, #855, .F. ) ;
#22075=CARTESIAN_POINT ( 'NONE',  ( 1.341640786499872284, 0.000000000000000000, 14.20000000000000107 ) ) ;
#22156=CARTESIAN_POINT ( 'NONE',  ( -1.341640786499875171, 0.000000000000000000, -11.80000000000000071 ) ) ;
#22307=CARTESIAN_POINT ( 'NONE',  ( -20.63749999999999929, 0.000000000000000000, -11.22499999999999787 ) ) ;
#22324=ORIENTED_EDGE ( 'NONE', *, *, #7281, .T. ) ;
#22389=AXIS2_PLACEMENT_3D ( 'NONE', #27493, #32471, #29993 ) ;
#22394=FACE_BOUND ( 'NONE', #12910, .T. ) ;
#22424=ORIENTED_EDGE ( 'NONE', *, *, #26085, .T. ) ;
#22453=VERTEX_POINT ( 'NONE', #23729 ) ;
#22663=SHAPE_REPRESENTATION_RELATIONSHIP ( 'NONE' , 'NONE' ,  #19821, #33925 ) ;
#22792=EDGE_CURVE ( 'NONE', #30850, #10045, #21120, .T. ) ;
#22813=AXIS2_PLACEMENT_3D ( 'NONE', #8972, #1314, #27830 ) ;
#22836=LINE ( 'NONE', #22307, #24665 ) ;
#22853=EDGE_LOOP ( 'NONE', ( #20689, #34571, #10150, #2172 ) ) ;
#22878=DIRECTION ( 'NONE',  ( 0.000000000000000000, 1.224646799147359124E-16, 1.000000000000000000 ) ) ;
#22963=ORIENTED_EDGE ( 'NONE', *, *, #29365, .F. ) ;
#22966=DIRECTION ( 'NONE',  ( 0.000000000000000000, 0.000000000000000000, -1.000000000000000000 ) ) ;
#22995=VECTOR ( 'NONE', #7534, 1000.000000000000000 ) ;
#23000=CARTESIAN_POINT ( 'NONE',  ( 0.000000000000000000, 0.000000000000000000, 0.000000000000000000 ) ) ;
#23083=CARTESIAN_POINT ( 'NONE',  ( 0.000000000000000000, 0.000000000000000000, 0.000000000000000000 ) ) ;
#23154=CARTESIAN_POINT ( 'NONE',  ( -1.341640786499875171, 0.000000000000000000, 0.000000000000000000 ) ) ;
#23169=DIRECTION ( 'NONE',  ( 1.000000000000000000, 0.000000000000000000, 0.000000000000000000 ) ) ;
#23208=CYLINDRICAL_SURFACE ( 'NONE', #27708, 14.77500000000000036 ) ;
#23218=VECTOR ( 'NONE', #33650, 1000.000000000000000 ) ;
#23243=VERTEX_POINT ( 'NONE', #25031 ) ;
#23359=EDGE_LOOP ( 'NONE', ( #22424, #15971, #17036, #32008 ) ) ;
#23390=EDGE_LOOP ( 'NONE', ( #30711, #379 ) ) ;
#23506=DIRECTION ( 'NONE',  ( 0.000000000000000000, 0.000000000000000000, -1.000000000000000000 ) ) ;
#23538=DIRECTION ( 'NONE',  ( 1.000000000000000000, 0.000000000000000000, 0.000000000000000000 ) ) ;
#23572=CARTESIAN_POINT ( 'NONE',  ( -20.63749999999999574, 0.000000000000000000, -16.00000000000000000 ) ) ;
#23633=CIRCLE ( 'NONE', #20242, 16.00000000000000000 ) ;
#23687=DIRECTION ( 'NONE',  ( 1.000000000000000000, 0.000000000000000000, 0.000000000000000000 ) ) ;
#23695=CIRCLE ( 'NONE', #21411, 14.20000000000000107 ) ;
#23704=ORIENTED_EDGE ( 'NONE', *, *, #13101, .T. ) ;
#23729=CARTESIAN_POINT ( 'NONE',  ( -7.700000000000000178, 0.000000000000000000, -9.999999999999998224 ) ) ;
#23774=DIRECTION ( 'NONE',  ( 0.000000000000000000, -1.000000000000000000, 0.000000000000000000 ) ) ;
#23878=VERTEX_POINT ( 'NONE', #16047 ) ;
#23892=DIRECTION ( 'NONE',  ( 0.000000000000000000, 0.000000000000000000, -1.000000000000000000 ) ) ;
#23901=CARTESIAN_POINT ( 'NONE',  ( -8.000000000000000000, 0.000000000000000000, 0.000000000000000000 ) ) ;
#23969=CARTESIAN_POINT ( 'NONE',  ( -7.700000000000000178, 0.000000000000000000, 0.000000000000000000 ) ) ;
#24067=CIRCLE ( 'NONE', #25213, 1.799999999999999600 ) ;
#24105=CARTESIAN_POINT ( 'NONE',  ( -20.63749999999999929, 0.000000000000000000, 0.000000000000000000 ) ) ;
#24156=CIRCLE ( 'NONE', #25871, 14.19999999999999929 ) ;
#24247=DIRECTION ( 'NONE',  ( 1.000000000000000000, 0.000000000000000000, 0.000000000000000000 ) ) ;
#24276=DIRECTION ( 'NONE',  ( 1.000000000000000000, 0.000000000000000000, 0.000000000000000000 ) ) ;
#24282=CARTESIAN_POINT ( 'NONE',  ( -0.2989565185775304723, 0.000000000000000000, 0.000000000000000000 ) ) ;
#24370=ORIENTED_EDGE ( 'NONE', *, *, #33517, .T. ) ;
#24411=FACE_OUTER_BOUND ( 'NONE', #14498, .T. ) ;
#24530=AXIS2_PLACEMENT_3D ( 'NONE', #23969, #7243, #15987 ) ;
#24533=ADVANCED_FACE ( 'NONE', ( #9903 ), #7044, .F. ) ;
#24622=CARTESIAN_POINT ( 'NONE',  ( 8.000000000000003553, 0.000000000000000000, 0.000000000000000000 ) ) ;
#24665=VECTOR ( 'NONE', #27989, 1000.000000000000000 ) ;
#24722=ORIENTED_EDGE ( 'NONE', *, *, #2757, .F. ) ;
#24847=CARTESIAN_POINT ( 'NONE',  ( -0.2989565185775304723, 0.000000000000000000, 14.77500000000000036 ) ) ;
#24905=AXIS2_PLACEMENT_3D ( 'NONE', #9958, #6922, #31488 ) ;
#24931=DIRECTION ( 'NONE',  ( -1.000000000000000000, -0.000000000000000000, -0.000000000000000000 ) ) ;
#24933=ORIENTED_EDGE ( 'NONE', *, *, #34970, .T. ) ;
#24966=EDGE_LOOP ( 'NONE', ( #5174, #21003 ) ) ;
#25031=CARTESIAN_POINT ( 'NONE',  ( 7.700000000000001954, 0.000000000000000000, -9.999999999999994671 ) ) ;
#25042=DIRECTION ( 'NONE',  ( 0.000000000000000000, 0.000000000000000000, -1.000000000000000000 ) ) ;
#25049=ORIENTED_EDGE ( 'NONE', *, *, #9092, .T. ) ;
#25090=CYLINDRICAL_SURFACE ( 'NONE', #27758, 11.22499999999999787 ) ;
#25094=PRODUCT_CONTEXT ( 'NONE', #7809, 'mechanical' ) ;
#25124=VERTEX_POINT ( 'NONE', #14558 ) ;
#25202=ORIENTED_EDGE ( 'NONE', *, *, #12158, .T. ) ;
#25213=AXIS2_PLACEMENT_3D ( 'NONE', #18580, #14640, #8742 ) ;
#25214=EDGE_CURVE ( 'NONE', #32572, #23243, #9811, .T. ) ;
#25242=FACE_OUTER_BOUND ( 'NONE', #13988, .T. ) ;
#25297=VECTOR ( 'NONE', #8309, 1000.000000000000000 ) ;
#25339=CARTESIAN_POINT ( 'NONE',  ( -8.000000000000000000, 1.809415645740213944E-15, 14.77499999999999858 ) ) ;
#25393=EDGE_LOOP ( 'NONE', ( #5395, #14679, #25049, #18840 ) ) ;
#25484=DIRECTION ( 'NONE',  ( 0.000000000000000000, 0.000000000000000000, 1.000000000000000000 ) ) ;
#25492=DIRECTION ( 'NONE',  ( 1.000000000000000000, 0.000000000000000000, 0.000000000000000000 ) ) ;
#25640=CARTESIAN_POINT ( 'NONE',  ( 7.700000000000000178, 0.000000000000000000, 0.000000000000000000 ) ) ;
#25661=ORIENTED_EDGE ( 'NONE', *, *, #25853, .F. ) ;
#25853=EDGE_CURVE ( 'NONE', #23878, #17976, #16693, .T. ) ;
#25871=AXIS2_PLACEMENT_3D ( 'NONE', #3674, #3330, #668 ) ;
#25875=ORIENTED_EDGE ( 'NONE', *, *, #277, .F. ) ;
#25917=DIRECTION ( 'NONE',  ( -1.000000000000000000, -0.000000000000000000, -0.000000000000000000 ) ) ;
#25952=EDGE_CURVE ( 'NONE', #21269, #12372, #26903, .T. ) ;
#25983=EDGE_CURVE ( 'NONE', #13790, #20178, #11008, .T. ) ;
#26003=DIRECTION ( 'NONE',  ( 1.000000000000000000, 0.000000000000000000, 0.000000000000000000 ) ) ;
#26066=EDGE_LOOP ( 'NONE', ( #21544, #30387, #22963, #3275 ) ) ;
#26085=EDGE_CURVE ( 'NONE', #16011, #29267, #10452, .T. ) ;
#26151=DIRECTION ( 'NONE',  ( 1.000000000000000000, 0.000000000000000000, 0.000000000000000000 ) ) ;
#26175=DIRECTION ( 'NONE',  ( 0.000000000000000000, -1.000000000000000000, 0.000000000000000000 ) ) ;
#26243=ORIENTED_EDGE ( 'NONE', *, *, #31141, .T. ) ;
#26364=VERTEX_POINT ( 'NONE', #22075 ) ;
#26372=CARTESIAN_POINT ( 'NONE',  ( -7.700000000000000178, 1.922695474661344271E-15, 15.69999999999999929 ) ) ;
#26380=DIRECTION ( 'NONE',  ( 1.000000000000000000, 0.000000000000000000, 0.000000000000000000 ) ) ;
#26398=AXIS2_PLACEMENT_3D ( 'NONE', #8186, #2846, #32227 ) ;
#26402=DIRECTION ( 'NONE',  ( 1.000000000000000000, 0.000000000000000000, 0.000000000000000000 ) ) ;
#26562=AXIS2_PLACEMENT_3D ( 'NONE', #7508, #31889, #2704 ) ;
#26575=FACE_OUTER_BOUND ( 'NONE', #35007, .T. ) ;
#26579=CARTESIAN_POINT ( 'NONE',  ( 0.000000000000000000, 0.000000000000000000, 0.000000000000000000 ) ) ;
#26607=CARTESIAN_POINT ( 'NONE',  ( -7.700000000000000178, 0.000000000000000000, -10.30000000000000071 ) ) ;
#26649=AXIS2_PLACEMENT_3D ( 'NONE', #20240, #14553, #11699 ) ;
#26826=DIRECTION ( 'NONE',  ( 0.000000000000000000, 0.000000000000000000, -1.000000000000000000 ) ) ;
#26888=CARTESIAN_POINT ( 'NONE',  ( 8.000000000000000000, 1.374666032042903655E-15, 11.22499999999999787 ) ) ;
#26903=CIRCLE ( 'NONE', #15008, 10.30000000000000071 ) ;
#26962=DIRECTION ( 'NONE',  ( 1.000000000000000000, 0.000000000000000000, 0.000000000000000000 ) ) ;
#26981=ADVANCED_FACE ( 'NONE', ( #29600 ), #31505, .T. ) ;
#27117=VECTOR ( 'NONE', #23169, 1000.000000000000000 ) ;
#27198=ORIENTED_EDGE ( 'NONE', *, *, #3593, .F. ) ;
#27229=DIRECTION ( 'NONE',  ( 0.000000000000000000, 0.000000000000000000, -1.000000000000000000 ) ) ;
#27301=DIRECTION ( 'NONE',  ( 0.000000000000000000, 0.000000000000000000, -1.000000000000000000 ) ) ;
#27303=ADVANCED_FACE ( 'NONE', ( #29562 ), #2314, .T. ) ;
#27493=CARTESIAN_POINT ( 'NONE',  ( -7.700000000000000178, 0.000000000000000000, 0.000000000000000000 ) ) ;
#27671=ADVANCED_FACE ( 'NONE', ( #1930 ), #4258, .T. ) ;
#27678=AXIS2_PLACEMENT_3D ( 'NONE', #9059, #19923, #6375 ) ;
#27708=AXIS2_PLACEMENT_3D ( 'NONE', #7155, #17704, #9667 ) ;
#27758=AXIS2_PLACEMENT_3D ( 'NONE', #27772, #30451, #22966 ) ;
#27772=CARTESIAN_POINT ( 'NONE',  ( -20.63749999999999929, 0.000000000000000000, 0.000000000000000000 ) ) ;
#27830=DIRECTION ( 'NONE',  ( 0.000000000000000000, 0.000000000000000000, -1.000000000000000000 ) ) ;
#27860=CIRCLE ( 'NONE', #13641, 11.80000000000000071 ) ;
#27989=DIRECTION ( 'NONE',  ( 1.000000000000000000, 0.000000000000000000, 0.000000000000000000 ) ) ;
#27995=CIRCLE ( 'NONE', #17785, 9.999999999999994671 ) ;
#28125=VERTEX_POINT ( 'NONE', #28430 ) ;
#28195=EDGE_LOOP ( 'NONE', ( #17381, #23704, #7994, #29823 ) ) ;
#28311=VECTOR ( 'NONE', #10404, 1000.000000000000000 ) ;
#28389=AXIS2_PLACEMENT_3D ( 'NONE', #24622, #264, #7731 ) ;
#28394=VECTOR ( 'NONE', #29049, 1000.000000000000000 ) ;
#28429=CARTESIAN_POINT ( 'NONE',  ( -20.63749999999999929, 0.000000000000000000, 0.000000000000000000 ) ) ;
#28430=CARTESIAN_POINT ( 'NONE',  ( -1.341640786499875171, 1.445083222993876839E-15, 11.80000000000000071 ) ) ;
#28442=ORIENTED_EDGE ( 'NONE', *, *, #21782, .F. ) ;
#28465=CIRCLE ( 'NONE', #21647, 11.22499999999999787 ) ;
#28498=EDGE_CURVE ( 'NONE', #29721, #12372, #34175, .T. ) ;
#28564=VERTEX_POINT ( 'NONE', #26888 ) ;
#28566=AXIS2_PLACEMENT_3D ( 'NONE', #26579, #2200, #13073 ) ;
#28587=DIRECTION ( 'NONE',  ( -1.000000000000000000, 0.000000000000000000, -0.000000000000000000 ) ) ;
#28652=DIRECTION ( 'NONE',  ( 0.000000000000000000, 0.000000000000000000, -1.000000000000000000 ) ) ;
#28756=FACE_BOUND ( 'NONE', #1632, .T. ) ;
#28762=CARTESIAN_POINT ( 'NONE',  ( 7.700000000000000178, 0.000000000000000000, -10.30000000000000071 ) ) ;
#28767=ORIENTED_EDGE ( 'NONE', *, *, #21011, .T. ) ;
#28774=DIRECTION ( 'NONE',  ( 1.000000000000000000, 0.000000000000000000, 0.000000000000000000 ) ) ;
#28823=CARTESIAN_POINT ( 'NONE',  ( 7.700000000000000178, 0.000000000000000000, 0.000000000000000000 ) ) ;
#28855=ADVANCED_FACE ( 'NONE', ( #12965 ), #20021, .T. ) ;
#29011=EDGE_LOOP ( 'NONE', ( #17079, #4194 ) ) ;
#29048=EDGE_CURVE ( 'NONE', #26364, #19238, #14145, .T. ) ;
#29049=DIRECTION ( 'NONE',  ( 1.000000000000000000, 0.000000000000000000, 0.000000000000000000 ) ) ;
#29069=CARTESIAN_POINT ( 'NONE',  ( 7.699999999999998401, 0.000000000000000000, 0.000000000000000000 ) ) ;
#29145=CIRCLE ( 'NONE', #13805, 9.999999999999998224 ) ;
#29146=AXIS2_PLACEMENT_3D ( 'NONE', #8232, #31906, #4852 ) ;
#29168=DIRECTION ( 'NONE',  ( 0.000000000000000000, 0.000000000000000000, -1.000000000000000000 ) ) ;
#29244=EDGE_CURVE ( 'NONE', #10045, #14714, #9838, .T. ) ;
#29267=VERTEX_POINT ( 'NONE', #29414 ) ;
#29276=AXIS2_PLACEMENT_3D ( 'NONE', #17638, #7086, #1759 ) ;
#29365=EDGE_CURVE ( 'NONE', #1870, #28564, #28465, .T. ) ;
#29393=CIRCLE ( 'NONE', #486, 11.22499999999999787 ) ;
#29414=CARTESIAN_POINT ( 'NONE',  ( -8.000000000000000000, 1.941065176648554701E-15, 15.69999999999999929 ) ) ;
#29502=EDGE_CURVE ( 'NONE', #32236, #15484, #17157, .T. ) ;
#29521=AXIS2_PLACEMENT_3D ( 'NONE', #8472, #2946, #9007 ) ;
#29562=FACE_OUTER_BOUND ( 'NONE', #26066, .T. ) ;
#29564=ADVANCED_FACE ( 'NONE', ( #33837 ), #17714, .T. ) ;
#29569=PRODUCT_DEFINITION_CONTEXT ( 'detailed design', #21229, 'design' ) ;
#29582=EDGE_CURVE ( 'NONE', #14714, #30633, #21113, .T. ) ;
#29600=FACE_OUTER_BOUND ( 'NONE', #11372, .T. ) ;
#29629=CARTESIAN_POINT ( 'NONE',  ( 8.000000000000000000, 0.000000000000000000, 0.000000000000000000 ) ) ;
#29662=FACE_OUTER_BOUND ( 'NONE', #18963, .T. ) ;
#29721=VERTEX_POINT ( 'NONE', #13012 ) ;
#29764=FACE_BOUND ( 'NONE', #17527, .T. ) ;
#29778=AXIS2_PLACEMENT_3D ( 'NONE', #2713, #24247, #32955 ) ;
#29819=DIRECTION ( 'NONE',  ( 0.000000000000000000, 0.000000000000000000, -1.000000000000000000 ) ) ;
#29823=ORIENTED_EDGE ( 'NONE', *, *, #34970, .F. ) ;
#29890=CIRCLE ( 'NONE', #20224, 10.30000000000000071 ) ;
#29907=DIRECTION ( 'NONE',  ( 0.000000000000000000, 0.000000000000000000, -1.000000000000000000 ) ) ;
#29965=EDGE_LOOP ( 'NONE', ( #21953, #10288, #1512, #5729 ) ) ;
#29993=DIRECTION ( 'NONE',  ( 0.000000000000000000, 0.000000000000000000, -1.000000000000000000 ) ) ;
#30053=ORIENTED_EDGE ( 'NONE', *, *, #14123, .T. ) ;
#30114=DIRECTION ( 'NONE',  ( -0.000000000000000000, 0.000000000000000000, 1.000000000000000000 ) ) ;
#30141=EDGE_LOOP ( 'NONE', ( #5668, #15183, #1474, #31872 ) ) ;
#30387=ORIENTED_EDGE ( 'NONE', *, *, #6778, .T. ) ;
#30423=CLOSED_SHELL ( 'NONE', ( #1949, #32732, #28855, #8, #11522, #10353, #31982, #8443, #29564, #34081, #27303, #12789, #6867, #9728, #34812, #13385, #27671, #24533, #10530, #21419, #26981, #16377, #20813, #20426, #13070, #21248, #4241, #12887 ) ) ;
#30443=AXIS2_PLACEMENT_3D ( 'NONE', #23083, #25917, #6851 ) ;
#30451=DIRECTION ( 'NONE',  ( 1.000000000000000000, 0.000000000000000000, 0.000000000000000000 ) ) ;
#30463=ORIENTED_EDGE ( 'NONE', *, *, #32484, .F. ) ;
#30582=DIRECTION ( 'NONE',  ( 1.000000000000000000, 0.000000000000000000, 0.000000000000000000 ) ) ;
#30633=VERTEX_POINT ( 'NONE', #22156 ) ;
#30658=AXIS2_PLACEMENT_3D ( 'NONE', #18437, #16116, #18100 ) ;
#30711=ORIENTED_EDGE ( 'NONE', *, *, #29365, .T. ) ;
#30812=VERTEX_POINT ( 'NONE', #3622 ) ;
#30824=CARTESIAN_POINT ( 'NONE',  ( -8.000000000000000000, 0.000000000000000000, 0.000000000000000000 ) ) ;
#30850=VERTEX_POINT ( 'NONE', #25339 ) ;
#30899=DIRECTION ( 'NONE',  ( 0.000000000000000000, 0.000000000000000000, -1.000000000000000000 ) ) ;
#31030=ORIENTED_EDGE ( 'NONE', *, *, #28498, .T. ) ;
#31098=ORIENTED_EDGE ( 'NONE', *, *, #29582, .T. ) ;
#31103=EDGE_CURVE ( 'NONE', #29721, #22453, #29145, .T. ) ;
#31141=EDGE_CURVE ( 'NONE', #9326, #25124, #10955, .T. ) ;
#31151=AXIS2_PLACEMENT_3D ( 'NONE', #2463, #13344, #32532 ) ;
#31178=CARTESIAN_POINT ( 'NONE',  ( -7.700000000000000178, 0.000000000000000000, 0.000000000000000000 ) ) ;
#31317=DIRECTION ( 'NONE',  ( 1.000000000000000000, 0.000000000000000000, 0.000000000000000000 ) ) ;
#31455=DIRECTION ( 'NONE',  ( 0.000000000000000000, 0.000000000000000000, -1.000000000000000000 ) ) ;
#31488=DIRECTION ( 'NONE',  ( 0.000000000000000000, 0.000000000000000000, -1.000000000000000000 ) ) ;
#31505=TOROIDAL_SURFACE ( 'NONE', #5350, 13.00000000000000000, 1.799999999999999822 ) ;
#31558=CIRCLE ( 'NONE', #14539, 14.77500000000000036 ) ;
#31592=FACE_BOUND ( 'NONE', #24966, .T. ) ;
#31660=CIRCLE ( 'NONE', #26562, 14.20000000000000107 ) ;
#31794=CARTESIAN_POINT ( 'NONE',  ( 8.000000000000003553, 1.261386203121773722E-15, 10.30000000000000071 ) ) ;
#31872=ORIENTED_EDGE ( 'NONE', *, *, #29244, .F. ) ;
#31889=DIRECTION ( 'NONE',  ( 1.000000000000000000, 0.000000000000000000, 0.000000000000000000 ) ) ;
#31906=DIRECTION ( 'NONE',  ( 1.000000000000000000, 0.000000000000000000, 0.000000000000000000 ) ) ;
#31969=CARTESIAN_POINT ( 'NONE',  ( 0.000000000000000000, 0.000000000000000000, 0.000000000000000000 ) ) ;
#31982=ADVANCED_FACE ( 'NONE', ( #19155 ), #3597, .T. ) ;
#32008=ORIENTED_EDGE ( 'NONE', *, *, #34316, .F. ) ;
#32048=ORIENTED_EDGE ( 'NONE', *, *, #31103, .F. ) ;
#32051=CIRCLE ( 'NONE', #29778, 11.80000000000000071 ) ;
#32121=CYLINDRICAL_SURFACE ( 'NONE', #2634, 9.999999999999996447 ) ;
#32227=DIRECTION ( 'NONE',  ( 0.000000000000000000, 0.000000000000000000, -1.000000000000000000 ) ) ;
#32236=VERTEX_POINT ( 'NONE', #7702 ) ;
#32262=CARTESIAN_POINT ( 'NONE',  ( 8.000000000000003553, 0.000000000000000000, 0.000000000000000000 ) ) ;
#32284=LINE ( 'NONE', #10766, #28311 ) ;
#32335=CARTESIAN_POINT ( 'NONE',  ( -8.000000000000000000, 0.000000000000000000, 0.000000000000000000 ) ) ;
#32354=DIRECTION ( 'NONE',  ( 1.000000000000000000, 0.000000000000000000, 0.000000000000000000 ) ) ;
#32471=DIRECTION ( 'NONE',  ( 1.000000000000000000, 0.000000000000000000, 0.000000000000000000 ) ) ;
#32474=( LENGTH_UNIT ( ) NAMED_UNIT ( * ) SI_UNIT ( .MILLI., .METRE. ) );
#32477=ORIENTED_EDGE ( 'NONE', *, *, #15862, .T. ) ;
#32484=EDGE_CURVE ( 'NONE', #30633, #28125, #32051, .T. ) ;
#32532=DIRECTION ( 'NONE',  ( 0.000000000000000000, 0.000000000000000000, -1.000000000000000000 ) ) ;
#32572=VERTEX_POINT ( 'NONE', #14472 ) ;
#32690=TOROIDAL_SURFACE ( 'NONE', #30443, 13.00000000000000000, 1.799999999999999822 ) ;
#32703=CIRCLE ( 'NONE', #12279, 15.69999999999999929 ) ;
#32732=ADVANCED_FACE ( 'NONE', ( #15516 ), #2151, .T. ) ;
#32839=DIRECTION ( 'NONE',  ( -1.000000000000000000, -0.000000000000000000, -0.000000000000000000 ) ) ;
#32841=ORIENTED_EDGE ( 'NONE', *, *, #3593, .T. ) ;
#32918=CARTESIAN_POINT ( 'NONE',  ( 0.000000000000000000, 1.592040838891559095E-15, -13.00000000000000000 ) ) ;
#32955=DIRECTION ( 'NONE',  ( 0.000000000000000000, 0.000000000000000000, -1.000000000000000000 ) ) ;
#32981=DIRECTION ( 'NONE',  ( 0.000000000000000000, 0.000000000000000000, -1.000000000000000000 ) ) ;
#33109=EDGE_LOOP ( 'NONE', ( #24722, #7929, #33958, #9902 ) ) ;
#33202=AXIS2_PLACEMENT_3D ( 'NONE', #6052, #8915, #11413 ) ;
#33333=ORIENTED_EDGE ( 'NONE', *, *, #20886, .F. ) ;
#33361=FACE_OUTER_BOUND ( 'NONE', #30141, .T. ) ;
#33384=DIRECTION ( 'NONE',  ( 1.000000000000000000, 0.000000000000000000, 0.000000000000000000 ) ) ;
#33497=DIRECTION ( 'NONE',  ( -1.000000000000000000, -0.000000000000000000, -0.000000000000000000 ) ) ;
#33507=ORIENTED_EDGE ( 'NONE', *, *, #13101, .F. ) ;
#33517=EDGE_CURVE ( 'NONE', #769, #19238, #24156, .T. ) ;
#33650=DIRECTION ( 'NONE',  ( 1.000000000000000000, 0.000000000000000000, 0.000000000000000000 ) ) ;
#33689=AXIS2_PLACEMENT_3D ( 'NONE', #8889, #6201, #3367 ) ;
#33697=CARTESIAN_POINT ( 'NONE',  ( -20.63749999999999574, 0.000000000000000000, -14.77500000000000036 ) ) ;
#33706=MANIFOLD_SOLID_BREP ( 'OuterRace', #30423 ) ;
#33766=EDGE_CURVE ( 'NONE', #10045, #30850, #34149, .T. ) ;
#33837=FACE_OUTER_BOUND ( 'NONE', #9525, .T. ) ;
#33925=ADVANCED_BREP_SHAPE_REPRESENTATION ( '', ( #33706, #28566 ), #17234 ) ;
#33947=EDGE_CURVE ( 'NONE', #9326, #23878, #11527, .T. ) ;
#33958=ORIENTED_EDGE ( 'NONE', *, *, #29244, .T. ) ;
#34061=DIRECTION ( 'NONE',  ( 1.000000000000000000, 0.000000000000000000, 0.000000000000000000 ) ) ;
#34067=DIRECTION ( 'NONE',  ( 0.000000000000000000, 0.000000000000000000, -1.000000000000000000 ) ) ;
#34081=ADVANCED_FACE ( 'NONE', ( #26575 ), #10746, .T. ) ;
#34086=ORIENTED_EDGE ( 'NONE', *, *, #17795, .F. ) ;
#34149=CIRCLE ( 'NONE', #8003, 14.77499999999999858 ) ;
#34158=ORIENTED_EDGE ( 'NONE', *, *, #25214, .F. ) ;
#34175=CIRCLE ( 'NONE', #18848, 0.3000000000000016542 ) ;
#34213=ORIENTED_EDGE ( 'NONE', *, *, #31103, .T. ) ;
#34222=DIRECTION ( 'NONE',  ( 0.000000000000000000, 0.000000000000000000, -1.000000000000000000 ) ) ;
#34316=EDGE_CURVE ( 'NONE', #16011, #20178, #5828, .T. ) ;
#34351=ORIENTED_EDGE ( 'NONE', *, *, #26085, .F. ) ;
#34540=CARTESIAN_POINT ( 'NONE',  ( -8.000000000000000000, 0.000000000000000000, 0.000000000000000000 ) ) ;
#34571=ORIENTED_EDGE ( 'NONE', *, *, #855, .T. ) ;
#34605=AXIS2_PLACEMENT_3D ( 'NONE', #32335, #19188, #26826 ) ;
#34611=EDGE_LOOP ( 'NONE', ( #6700, #15536, #19995, #21573 ) ) ;
#34624=AXIS2_PLACEMENT_3D ( 'NONE', #31969, #7940, #7578 ) ;
#34720=DIRECTION ( 'NONE',  ( 1.000000000000000000, 0.000000000000000000, 0.000000000000000000 ) ) ;
#34804=DIRECTION ( 'NONE',  ( 0.000000000000000000, 0.000000000000000000, -1.000000000000000000 ) ) ;
#34806=FACE_OUTER_BOUND ( 'NONE', #12767, .T. ) ;
#34812=ADVANCED_FACE ( 'NONE', ( #13336 ), #4946, .T. ) ;
#34824=AXIS2_PLACEMENT_3D ( 'NONE', #29069, #26402, #34067 ) ;
#34877=AXIS2_PLACEMENT_3D ( 'NONE', #31178, #34720, #10158 ) ;
#34882=EDGE_CURVE ( 'NONE', #17435, #30812, #10908, .T. ) ;
#34899=AXIS2_PLACEMENT_3D ( 'NONE', #34540, #26003, #23506 ) ;
#34926=ORIENTED_EDGE ( 'NONE', *, *, #12607, .F. ) ;
#34970=EDGE_CURVE ( 'NONE', #30812, #23243, #27995, .T. ) ;
#35007=EDGE_LOOP ( 'NONE', ( #11285, #9495, #30463, #1061 ) ) ;
#35032=AXIS2_PLACEMENT_3D ( 'NONE', #32918, #20420, #3197 ) ;
#35269=COLOUR_RGB('Grey',0.48,0.52,0.57);
#35270=FILL_AREA_STYLE_COLOUR('',#35269);
#35271=FILL_AREA_STYLE('',(#35270));
#35272=SURFACE_STYLE_FILL_AREA(#35271);
#35273=SURFACE_SIDE_STYLE('',(#35272));
#35274=SURFACE_STYLE_USAGE(.BOTH.,#35273);
#35275=PRESENTATION_STYLE_ASSIGNMENT((#35274));
ENDSEC;
END-ISO-10303-21;
